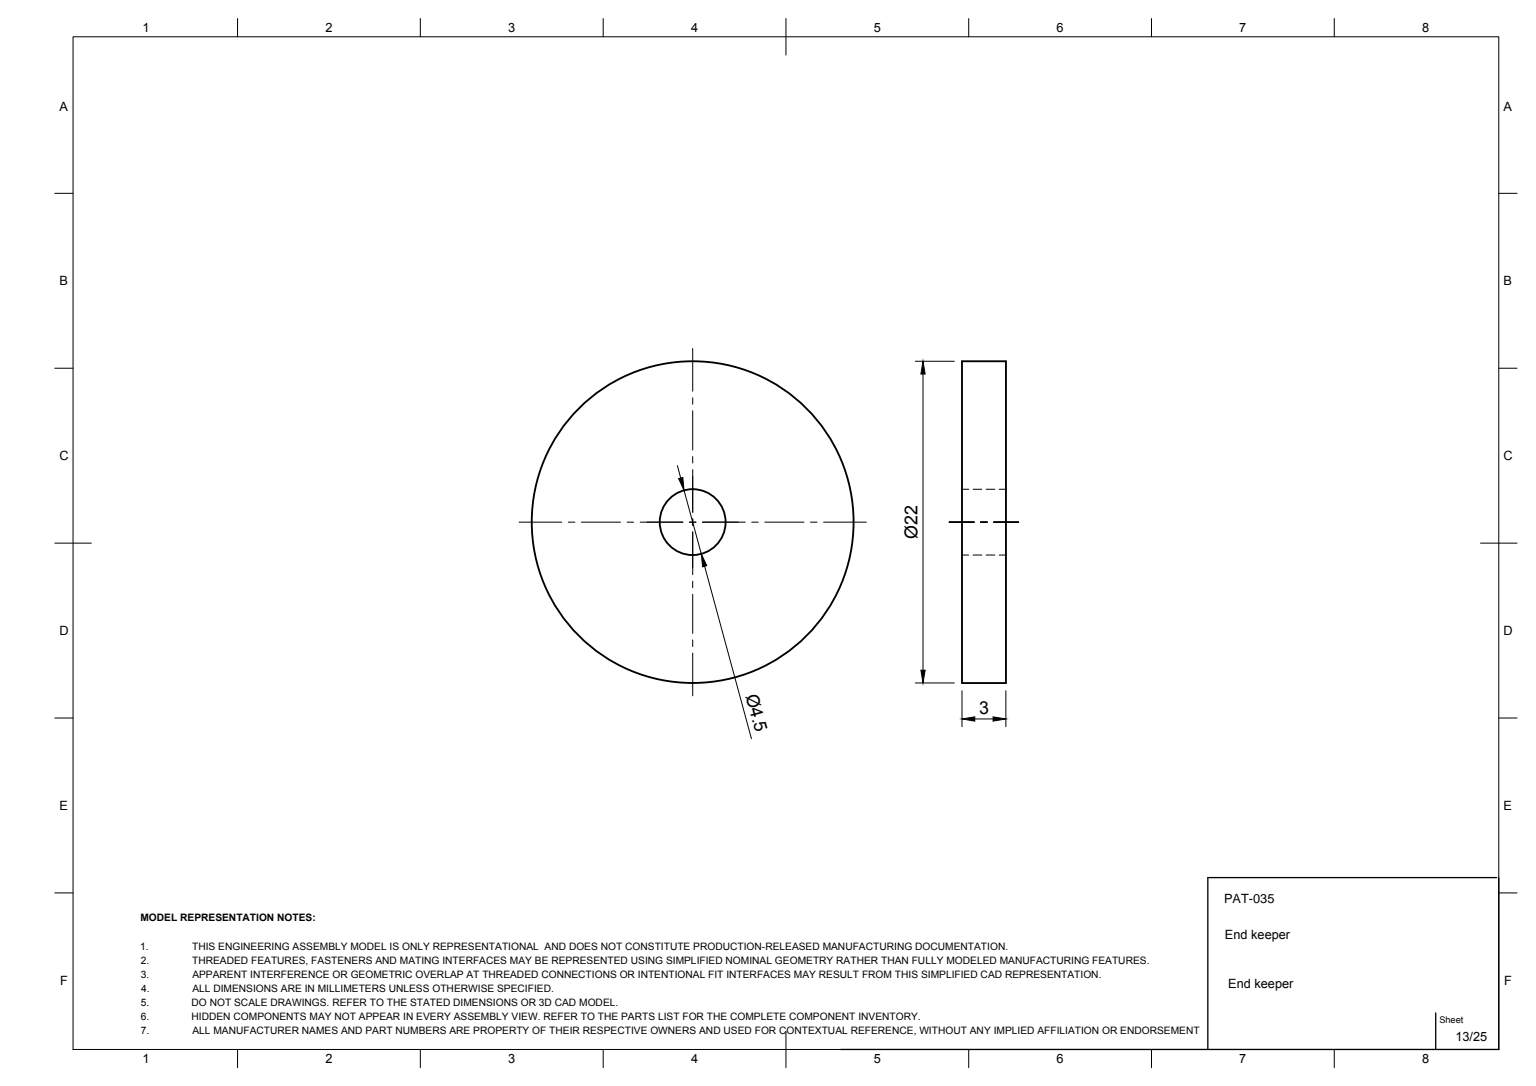
ISO-10303-21;
HEADER;
/* Generated by software containing ST-Developer
 * from STEP Tools, Inc. (www.steptools.com) 
 */

FILE_DESCRIPTION(
/* description */ ('Five-roller gravity conveyor'),
/* implementation_level */ '2;1');

FILE_NAME(
/* name */ 'End keeper.step',
/* time_stamp */ '2026-10-29T15:36:43-07:00',
/* author */ (''),
/* organization */ (''),
/* preprocessor_version */ 'ST-DEVELOPER v20.2',
/* originating_system */ 'Autodesk Translation Framework v15.17.0.0',
/* authorisation */ '');

FILE_SCHEMA (('AUTOMOTIVE_DESIGN { 1 0 10303 214 3 1 1 }'));
ENDSEC;

DATA;
#10=MECHANICAL_DESIGN_GEOMETRIC_PRESENTATION_REPRESENTATION('',(#331),#7806);
#287=SHAPE_REPRESENTATION_RELATIONSHIP('SRR','None',#7925,#305);
#305=ADVANCED_BREP_SHAPE_REPRESENTATION('',(#356),#7798);
#331=STYLED_ITEM('',(#8105),#356);
#356=MANIFOLD_SOLID_BREP('Body1',#4219);
#391=FACE_BOUND('',#1097,.T.);
#392=FACE_BOUND('',#1099,.T.);
#544=CIRCLE('',#4754,0.225);
#545=CIRCLE('',#4755,0.225);
#546=CIRCLE('',#4757,1.1);
#547=CIRCLE('',#4758,1.1);
#629=CYLINDRICAL_SURFACE('',#4753,0.225);
#630=CYLINDRICAL_SURFACE('',#4756,1.1);
#833=FACE_OUTER_BOUND('',#1094,.T.);
#834=FACE_OUTER_BOUND('',#1095,.T.);
#835=FACE_OUTER_BOUND('',#1096,.T.);
#836=FACE_OUTER_BOUND('',#1098,.T.);
#1094=EDGE_LOOP('',(#3632,#3633,#3634,#3635));
#1095=EDGE_LOOP('',(#3636,#3637,#3638,#3639));
#1096=EDGE_LOOP('',(#3640));
#1097=EDGE_LOOP('',(#3641));
#1098=EDGE_LOOP('',(#3642));
#1099=EDGE_LOOP('',(#3643));
#1471=LINE('',#7500,#1812);
#1472=LINE('',#7506,#1813);
#1812=VECTOR('',#5863,0.225);
#1813=VECTOR('',#5870,1.1);
#2158=VERTEX_POINT('',#7497);
#2159=VERTEX_POINT('',#7499);
#2160=VERTEX_POINT('',#7503);
#2161=VERTEX_POINT('',#7505);
#2659=EDGE_CURVE('',#2158,#2158,#544,.T.);
#2660=EDGE_CURVE('',#2158,#2159,#1471,.T.);
#2661=EDGE_CURVE('',#2159,#2159,#545,.T.);
#2662=EDGE_CURVE('',#2160,#2160,#546,.T.);
#2663=EDGE_CURVE('',#2160,#2161,#1472,.T.);
#2664=EDGE_CURVE('',#2161,#2161,#547,.T.);
#3632=ORIENTED_EDGE('',*,*,#2659,.F.);
#3633=ORIENTED_EDGE('',*,*,#2660,.T.);
#3634=ORIENTED_EDGE('',*,*,#2661,.T.);
#3635=ORIENTED_EDGE('',*,*,#2660,.F.);
#3636=ORIENTED_EDGE('',*,*,#2662,.F.);
#3637=ORIENTED_EDGE('',*,*,#2663,.T.);
#3638=ORIENTED_EDGE('',*,*,#2664,.T.);
#3639=ORIENTED_EDGE('',*,*,#2663,.F.);
#3640=ORIENTED_EDGE('',*,*,#2662,.T.);
#3641=ORIENTED_EDGE('',*,*,#2659,.T.);
#3642=ORIENTED_EDGE('',*,*,#2664,.F.);
#3643=ORIENTED_EDGE('',*,*,#2661,.F.);
#3943=PLANE('',#4759);
#3944=PLANE('',#4760);
#4148=ADVANCED_FACE('',(#833),#629,.F.);
#4149=ADVANCED_FACE('',(#834),#630,.T.);
#4150=ADVANCED_FACE('',(#835,#391),#3943,.T.);
#4151=ADVANCED_FACE('',(#836,#392),#3944,.F.);
#4219=CLOSED_SHELL('',(#4148,#4149,#4150,#4151));
#4752=AXIS2_PLACEMENT_3D('',#7495,#5857,#5858);
#4753=AXIS2_PLACEMENT_3D('',#7496,#5859,#5860);
#4754=AXIS2_PLACEMENT_3D('',#7498,#5861,#5862);
#4755=AXIS2_PLACEMENT_3D('',#7501,#5864,#5865);
#4756=AXIS2_PLACEMENT_3D('',#7502,#5866,#5867);
#4757=AXIS2_PLACEMENT_3D('',#7504,#5868,#5869);
#4758=AXIS2_PLACEMENT_3D('',#7507,#5871,#5872);
#4759=AXIS2_PLACEMENT_3D('',#7508,#5873,#5874);
#4760=AXIS2_PLACEMENT_3D('',#7509,#5875,#5876);
#5857=DIRECTION('axis',(0.,0.,1.));
#5858=DIRECTION('refdir',(1.,0.,0.));
#5859=DIRECTION('center_axis',(0.,1.,0.));
#5860=DIRECTION('ref_axis',(1.,0.,0.));
#5861=DIRECTION('center_axis',(0.,-1.,0.));
#5862=DIRECTION('ref_axis',(1.,0.,0.));
#5863=DIRECTION('',(0.,-1.,0.));
#5864=DIRECTION('center_axis',(0.,-1.,0.));
#5865=DIRECTION('ref_axis',(1.,0.,0.));
#5866=DIRECTION('center_axis',(0.,1.,0.));
#5867=DIRECTION('ref_axis',(1.,0.,0.));
#5868=DIRECTION('center_axis',(0.,1.,0.));
#5869=DIRECTION('ref_axis',(1.,0.,0.));
#5870=DIRECTION('',(0.,-1.,0.));
#5871=DIRECTION('center_axis',(0.,1.,0.));
#5872=DIRECTION('ref_axis',(1.,0.,0.));
#5873=DIRECTION('center_axis',(0.,1.,0.));
#5874=DIRECTION('ref_axis',(1.,0.,0.));
#5875=DIRECTION('center_axis',(0.,1.,0.));
#5876=DIRECTION('ref_axis',(1.,0.,0.));
#7495=CARTESIAN_POINT('',(0.,0.,0.));
#7496=CARTESIAN_POINT('Origin',(0.,-2.8,4.5));
#7497=CARTESIAN_POINT('',(-0.225,-2.5,4.5));
#7498=CARTESIAN_POINT('Origin',(0.,-2.5,4.5));
#7499=CARTESIAN_POINT('',(-0.225,-2.8,4.5));
#7500=CARTESIAN_POINT('',(-0.225,-2.8,4.5));
#7501=CARTESIAN_POINT('Origin',(0.,-2.8,4.5));
#7502=CARTESIAN_POINT('Origin',(0.,-2.8,4.5));
#7503=CARTESIAN_POINT('',(-1.1,-2.5,4.5));
#7504=CARTESIAN_POINT('Origin',(0.,-2.5,4.5));
#7505=CARTESIAN_POINT('',(-1.1,-2.8,4.5));
#7506=CARTESIAN_POINT('',(-1.1,-2.8,4.5));
#7507=CARTESIAN_POINT('Origin',(0.,-2.8,4.5));
#7508=CARTESIAN_POINT('Origin',(0.,-2.5,4.5));
#7509=CARTESIAN_POINT('Origin',(0.,-2.8,4.5));
#7774=UNCERTAINTY_MEASURE_WITH_UNIT(LENGTH_MEASURE(0.001),#7807,
'DISTANCE_ACCURACY_VALUE',
'Maximum model space distance between geometric entities at asserted c
onnectivities');
#7782=UNCERTAINTY_MEASURE_WITH_UNIT(LENGTH_MEASURE(0.001),#7807,
'DISTANCE_ACCURACY_VALUE',
'Maximum model space distance between geometric entities at asserted c
onnectivities');
#7798=(
GEOMETRIC_REPRESENTATION_CONTEXT(3)
GLOBAL_UNCERTAINTY_ASSIGNED_CONTEXT((#7774))
GLOBAL_UNIT_ASSIGNED_CONTEXT((#7807,#7809,#7810))
REPRESENTATION_CONTEXT('','3D')
);
#7806=(
GEOMETRIC_REPRESENTATION_CONTEXT(3)
GLOBAL_UNCERTAINTY_ASSIGNED_CONTEXT((#7782))
GLOBAL_UNIT_ASSIGNED_CONTEXT((#7807,#7809,#7810))
REPRESENTATION_CONTEXT('','3D')
);
#7807=(
LENGTH_UNIT()
NAMED_UNIT(*)
SI_UNIT(.CENTI.,.METRE.)
);
#7809=(
NAMED_UNIT(*)
PLANE_ANGLE_UNIT()
SI_UNIT($,.RADIAN.)
);
#7810=(
NAMED_UNIT(*)
SI_UNIT($,.STERADIAN.)
SOLID_ANGLE_UNIT()
);
#7826=SHAPE_DEFINITION_REPRESENTATION(#7854,#7925);
#7854=PRODUCT_DEFINITION_SHAPE('',$,#7949);
#7925=SHAPE_REPRESENTATION('',(#4752),#7798);
#7933=PRODUCT_DEFINITION_CONTEXT('part definition',#8004,'design');
#7949=PRODUCT_DEFINITION('End keeper','End keeper',#7972,#7933);
#7972=PRODUCT_DEFINITION_FORMATION('',$,#8021);
#8004=APPLICATION_CONTEXT(
'Core Data for Automotive Mechanical Design Process');
#8005=PRODUCT_CONTEXT('part definition',#8004,'mechanical');
#8021=PRODUCT('End keeper','End keeper','End keeper',(#8005));
#8099=COLOUR_RGB('Off White',0.89,0.88,0.83);
#8100=FILL_AREA_STYLE_COLOUR('',#8099);
#8101=FILL_AREA_STYLE('',(#8100));
#8102=SURFACE_STYLE_FILL_AREA(#8101);
#8103=SURFACE_SIDE_STYLE('',(#8102));
#8104=SURFACE_STYLE_USAGE(.BOTH.,#8103);
#8105=PRESENTATION_STYLE_ASSIGNMENT((#8104));
ENDSEC;
END-ISO-10303-21;
